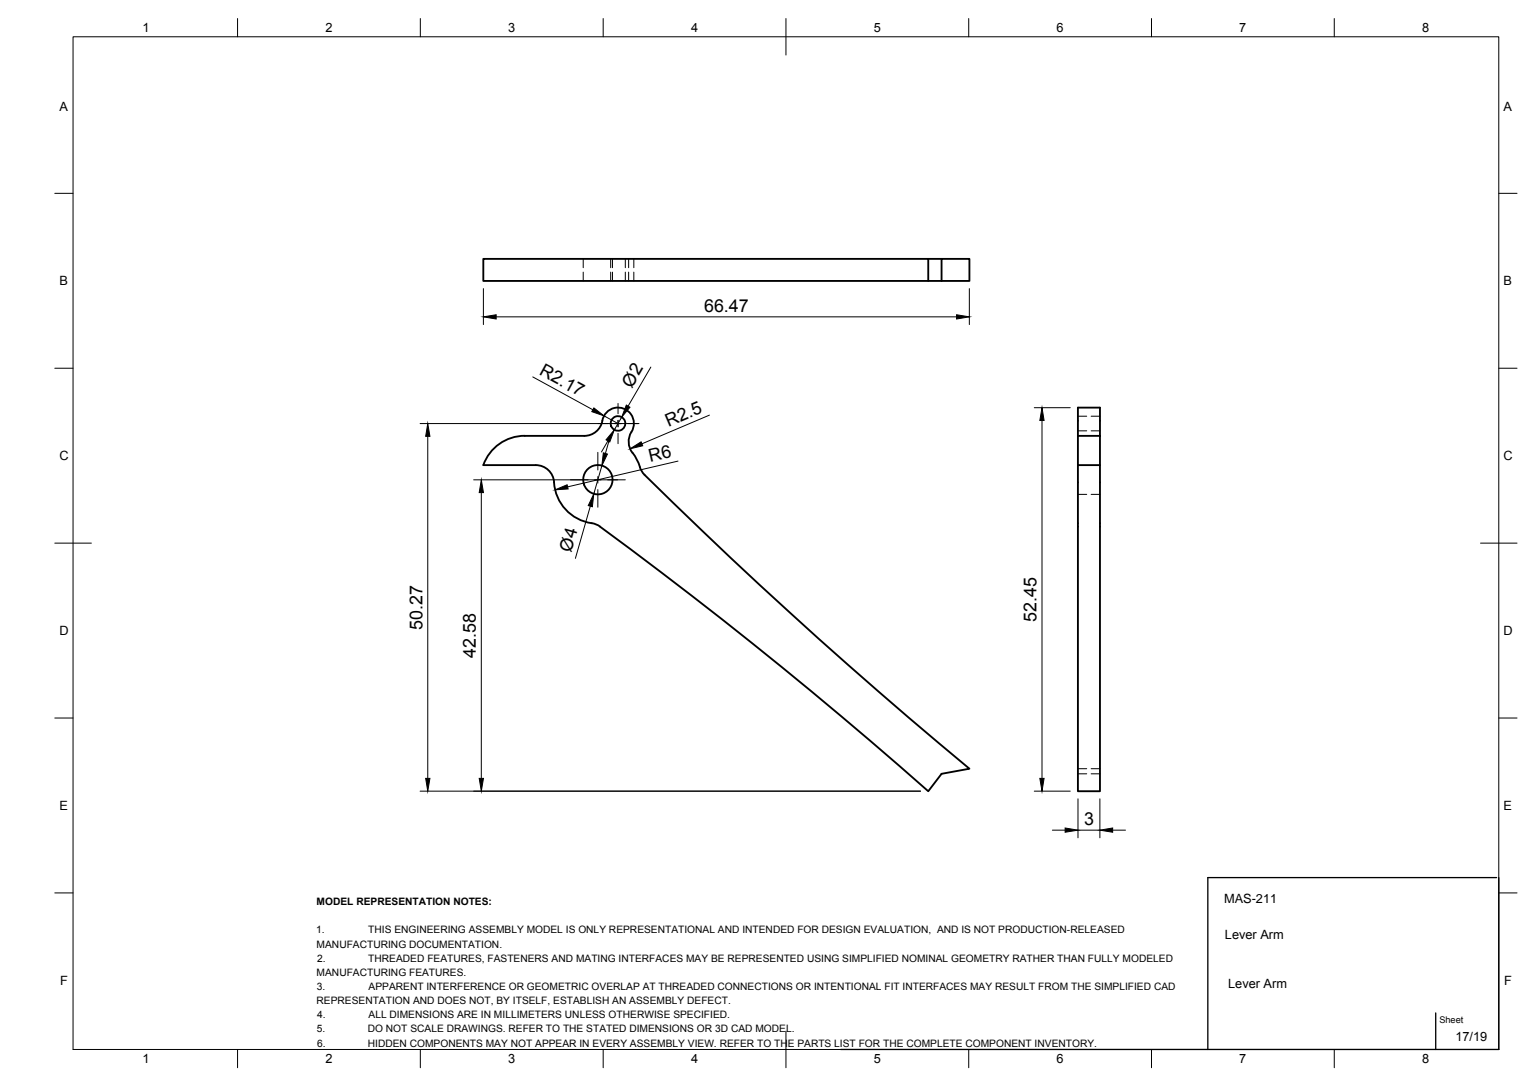
ISO-10303-21;
HEADER;
FILE_DESCRIPTION(
 (''),
 '2;1');
FILE_NAME ( 'Lever Arm.step', '2026-10-05T20:07:59+06:00', ( '' ), ( '' ), 'STEP AP214', 'Unspecified', '' );
FILE_SCHEMA (('AUTOMOTIVE_DESIGN { 1 0 10303 214 3 1 1 }'));
ENDSEC;
DATA;
#10=MECHANICAL_DESIGN_GEOMETRIC_PRESENTATION_REPRESENTATION('',(#335),#196741);
#69=(
BOUNDED_SURFACE()
B_SPLINE_SURFACE(2,1,((#194720,#194721),(#194722,#194723),(#194724,#194725)),
 .UNSPECIFIED.,.F.,.F.,.F.)
B_SPLINE_SURFACE_WITH_KNOTS((3,3),(2,2),(-66.4194892732842,-6.49328858992507),
(0.,0.36),.UNSPECIFIED.)
GEOMETRIC_REPRESENTATION_ITEM()
RATIONAL_B_SPLINE_SURFACE(((1.,1.),(0.999060551236508,0.999060551236508),
(1.,1.)))
REPRESENTATION_ITEM('')
SURFACE()
) ;
#70=(
BOUNDED_SURFACE()
B_SPLINE_SURFACE(2,1,((#194797,#194798),(#194799,#194800),(#194801,#194802)),
 .UNSPECIFIED.,.F.,.F.,.F.)
B_SPLINE_SURFACE_WITH_KNOTS((3,3),(2,2),(47.1134450647953,104.780247485259),
(0.,0.36),.UNSPECIFIED.)
GEOMETRIC_REPRESENTATION_ITEM()
RATIONAL_B_SPLINE_SURFACE(((1.,1.),(0.998981521269156,0.998981521269156),
(1.,1.)))
REPRESENTATION_ITEM('')
SURFACE()
) ;
#335=STYLED_ITEM('',(#196765),#354) ;
#354=MANIFOLD_SOLID_BREP('Lever Arm',#8731) ;
#410=PLANE('',#9042) ;
#411=PLANE('',#9060) ;
#412=PLANE('',#9064) ;
#413=PLANE('',#9076) ;
#414=PLANE('',#9083) ;
#415=PLANE('',#9084) ;
#590=FACE_BOUND('',#1605,.T.) ;
#591=FACE_BOUND('',#1606,.T.) ;
#592=FACE_BOUND('',#1608,.T.) ;
#593=FACE_BOUND('',#1609,.T.) ;
#711=CIRCLE('',#9043,691.195967278452) ;
#712=CIRCLE('',#9044,691.195967278452) ;
#713=CIRCLE('',#9046,2.49999999999962) ;
#714=CIRCLE('',#9047,2.49999999999962) ;
#715=CIRCLE('',#9049,5.99999999999934) ;
#716=CIRCLE('',#9050,5.99999999999934) ;
#717=CIRCLE('',#9052,2.50000000000002) ;
#718=CIRCLE('',#9053,2.50000000000002) ;
#719=CIRCLE('',#9055,2.17161327008905) ;
#720=CIRCLE('',#9056,2.17161327008905) ;
#721=CIRCLE('',#9058,2.50000000000002) ;
#722=CIRCLE('',#9059,2.50000000000002) ;
#723=CIRCLE('',#9062,6.00000000000005) ;
#724=CIRCLE('',#9063,6.00000000000005) ;
#725=CIRCLE('',#9066,2.49999999999997) ;
#726=CIRCLE('',#9067,2.49999999999997) ;
#727=CIRCLE('',#9069,6.00000000000009) ;
#728=CIRCLE('',#9070,6.00000000000009) ;
#729=CIRCLE('',#9072,2.50000000000032) ;
#730=CIRCLE('',#9073,2.50000000000032) ;
#731=CIRCLE('',#9074,638.804590655714) ;
#732=CIRCLE('',#9075,638.804590655714) ;
#733=CIRCLE('',#9078,2.00000000000002) ;
#734=CIRCLE('',#9079,2.00000000000002) ;
#735=CIRCLE('',#9081,1.) ;
#736=CIRCLE('',#9082,1.) ;
#1078=FACE_OUTER_BOUND('',#1587,.T.) ;
#1079=FACE_OUTER_BOUND('',#1588,.T.) ;
#1080=FACE_OUTER_BOUND('',#1589,.T.) ;
#1081=FACE_OUTER_BOUND('',#1590,.T.) ;
#1082=FACE_OUTER_BOUND('',#1591,.T.) ;
#1083=FACE_OUTER_BOUND('',#1592,.T.) ;
#1084=FACE_OUTER_BOUND('',#1593,.T.) ;
#1085=FACE_OUTER_BOUND('',#1594,.T.) ;
#1086=FACE_OUTER_BOUND('',#1595,.T.) ;
#1087=FACE_OUTER_BOUND('',#1596,.T.) ;
#1088=FACE_OUTER_BOUND('',#1597,.T.) ;
#1089=FACE_OUTER_BOUND('',#1598,.T.) ;
#1090=FACE_OUTER_BOUND('',#1599,.T.) ;
#1091=FACE_OUTER_BOUND('',#1600,.T.) ;
#1092=FACE_OUTER_BOUND('',#1601,.T.) ;
#1093=FACE_OUTER_BOUND('',#1602,.T.) ;
#1094=FACE_OUTER_BOUND('',#1603,.T.) ;
#1095=FACE_OUTER_BOUND('',#1604,.T.) ;
#1096=FACE_OUTER_BOUND('',#1607,.T.) ;
#1587=EDGE_LOOP('',(#6656,#6657,#6658,#6659)) ;
#1588=EDGE_LOOP('',(#6660,#6661,#6662,#6663)) ;
#1589=EDGE_LOOP('',(#6664,#6665,#6666,#6667)) ;
#1590=EDGE_LOOP('',(#6668,#6669,#6670,#6671)) ;
#1591=EDGE_LOOP('',(#6672,#6673,#6674,#6675)) ;
#1592=EDGE_LOOP('',(#6676,#6677,#6678,#6679)) ;
#1593=EDGE_LOOP('',(#6680,#6681,#6682,#6683)) ;
#1594=EDGE_LOOP('',(#6684,#6685,#6686,#6687)) ;
#1595=EDGE_LOOP('',(#6688,#6689,#6690,#6691)) ;
#1596=EDGE_LOOP('',(#6692,#6693,#6694,#6695)) ;
#1597=EDGE_LOOP('',(#6696,#6697,#6698,#6699)) ;
#1598=EDGE_LOOP('',(#6700,#6701,#6702,#6703)) ;
#1599=EDGE_LOOP('',(#6704,#6705,#6706,#6707)) ;
#1600=EDGE_LOOP('',(#6708,#6709,#6710,#6711)) ;
#1601=EDGE_LOOP('',(#6712,#6713,#6714,#6715)) ;
#1602=EDGE_LOOP('',(#6716,#6717,#6718,#6719)) ;
#1603=EDGE_LOOP('',(#6720,#6721,#6722,#6723)) ;
#1604=EDGE_LOOP('',(#6724,#6725,#6726,#6727,#6728,#6729,#6730,#6731,#6732,
#6733,#6734,#6735,#6736,#6737,#6738)) ;
#1605=EDGE_LOOP('',(#6739)) ;
#1606=EDGE_LOOP('',(#6740)) ;
#1607=EDGE_LOOP('',(#6741,#6742,#6743,#6744,#6745,#6746,#6747,#6748,#6749,
#6750,#6751,#6752,#6753,#6754,#6755)) ;
#1608=EDGE_LOOP('',(#6756)) ;
#1609=EDGE_LOOP('',(#6757)) ;
#2054=LINE('',#194714,#2757) ;
#2055=LINE('',#194716,#2758) ;
#2056=LINE('',#194718,#2759) ;
#2057=LINE('',#194719,#2760) ;
#2058=LINE('',#194729,#2761) ;
#2059=LINE('',#194735,#2762) ;
#2060=LINE('',#194741,#2763) ;
#2061=LINE('',#194747,#2764) ;
#2062=LINE('',#194753,#2765) ;
#2063=LINE('',#194759,#2766) ;
#2064=LINE('',#194763,#2767) ;
#2065=LINE('',#194765,#2768) ;
#2066=LINE('',#194766,#2769) ;
#2067=LINE('',#194771,#2770) ;
#2068=LINE('',#194775,#2771) ;
#2069=LINE('',#194777,#2772) ;
#2070=LINE('',#194778,#2773) ;
#2071=LINE('',#194783,#2774) ;
#2072=LINE('',#194789,#2775) ;
#2073=LINE('',#194795,#2776) ;
#2074=LINE('',#194806,#2777) ;
#2075=LINE('',#194809,#2778) ;
#2076=LINE('',#194810,#2779) ;
#2077=LINE('',#194815,#2780) ;
#2078=LINE('',#194821,#2781) ;
#2757=VECTOR('',#10240,10.) ;
#2758=VECTOR('',#10241,10.) ;
#2759=VECTOR('',#10242,10.) ;
#2760=VECTOR('',#10243,10.) ;
#2761=VECTOR('',#10246,10.) ;
#2762=VECTOR('',#10253,10.) ;
#2763=VECTOR('',#10260,10.) ;
#2764=VECTOR('',#10267,10.) ;
#2765=VECTOR('',#10274,10.) ;
#2766=VECTOR('',#10281,10.) ;
#2767=VECTOR('',#10286,10.) ;
#2768=VECTOR('',#10287,10.) ;
#2769=VECTOR('',#10288,10.) ;
#2770=VECTOR('',#10293,10.) ;
#2771=VECTOR('',#10298,10.) ;
#2772=VECTOR('',#10299,10.) ;
#2773=VECTOR('',#10300,10.) ;
#2774=VECTOR('',#10305,10.) ;
#2775=VECTOR('',#10312,10.) ;
#2776=VECTOR('',#10319,10.) ;
#2777=VECTOR('',#10324,10.) ;
#2778=VECTOR('',#10329,10.) ;
#2779=VECTOR('',#10330,10.) ;
#2780=VECTOR('',#10335,2.00000000000001) ;
#2781=VECTOR('',#10342,0.999999999999978) ;
#3804=VERTEX_POINT('',#194712) ;
#3805=VERTEX_POINT('',#194713) ;
#3806=VERTEX_POINT('',#194715) ;
#3807=VERTEX_POINT('',#194717) ;
#3808=VERTEX_POINT('',#194726) ;
#3809=VERTEX_POINT('',#194728) ;
#3810=VERTEX_POINT('',#194732) ;
#3811=VERTEX_POINT('',#194734) ;
#3812=VERTEX_POINT('',#194738) ;
#3813=VERTEX_POINT('',#194740) ;
#3814=VERTEX_POINT('',#194744) ;
#3815=VERTEX_POINT('',#194746) ;
#3816=VERTEX_POINT('',#194750) ;
#3817=VERTEX_POINT('',#194752) ;
#3818=VERTEX_POINT('',#194756) ;
#3819=VERTEX_POINT('',#194758) ;
#3820=VERTEX_POINT('',#194762) ;
#3821=VERTEX_POINT('',#194764) ;
#3822=VERTEX_POINT('',#194768) ;
#3823=VERTEX_POINT('',#194770) ;
#3824=VERTEX_POINT('',#194774) ;
#3825=VERTEX_POINT('',#194776) ;
#3826=VERTEX_POINT('',#194780) ;
#3827=VERTEX_POINT('',#194782) ;
#3828=VERTEX_POINT('',#194786) ;
#3829=VERTEX_POINT('',#194788) ;
#3830=VERTEX_POINT('',#194792) ;
#3831=VERTEX_POINT('',#194794) ;
#3832=VERTEX_POINT('',#194803) ;
#3833=VERTEX_POINT('',#194805) ;
#3834=VERTEX_POINT('',#194812) ;
#3835=VERTEX_POINT('',#194814) ;
#3836=VERTEX_POINT('',#194818) ;
#3837=VERTEX_POINT('',#194820) ;
#4836=EDGE_CURVE('',#3804,#3805,#2054,.T.) ;
#4837=EDGE_CURVE('',#3805,#3806,#2055,.T.) ;
#4838=EDGE_CURVE('',#3807,#3806,#2056,.T.) ;
#4839=EDGE_CURVE('',#3804,#3807,#2057,.T.) ;
#4840=EDGE_CURVE('',#3805,#3808,#711,.T.) ;
#4841=EDGE_CURVE('',#3808,#3809,#2058,.T.) ;
#4842=EDGE_CURVE('',#3806,#3809,#712,.T.) ;
#4843=EDGE_CURVE('',#3808,#3810,#713,.T.) ;
#4844=EDGE_CURVE('',#3810,#3811,#2059,.T.) ;
#4845=EDGE_CURVE('',#3809,#3811,#714,.T.) ;
#4846=EDGE_CURVE('',#3810,#3812,#715,.T.) ;
#4847=EDGE_CURVE('',#3812,#3813,#2060,.T.) ;
#4848=EDGE_CURVE('',#3811,#3813,#716,.T.) ;
#4849=EDGE_CURVE('',#3812,#3814,#717,.T.) ;
#4850=EDGE_CURVE('',#3814,#3815,#2061,.T.) ;
#4851=EDGE_CURVE('',#3813,#3815,#718,.T.) ;
#4852=EDGE_CURVE('',#3814,#3816,#719,.T.) ;
#4853=EDGE_CURVE('',#3816,#3817,#2062,.T.) ;
#4854=EDGE_CURVE('',#3815,#3817,#720,.T.) ;
#4855=EDGE_CURVE('',#3816,#3818,#721,.T.) ;
#4856=EDGE_CURVE('',#3818,#3819,#2063,.T.) ;
#4857=EDGE_CURVE('',#3817,#3819,#722,.T.) ;
#4858=EDGE_CURVE('',#3818,#3820,#2064,.T.) ;
#4859=EDGE_CURVE('',#3820,#3821,#2065,.T.) ;
#4860=EDGE_CURVE('',#3819,#3821,#2066,.T.) ;
#4861=EDGE_CURVE('',#3820,#3822,#723,.T.) ;
#4862=EDGE_CURVE('',#3822,#3823,#2067,.T.) ;
#4863=EDGE_CURVE('',#3821,#3823,#724,.T.) ;
#4864=EDGE_CURVE('',#3822,#3824,#2068,.T.) ;
#4865=EDGE_CURVE('',#3824,#3825,#2069,.T.) ;
#4866=EDGE_CURVE('',#3823,#3825,#2070,.T.) ;
#4867=EDGE_CURVE('',#3824,#3826,#725,.T.) ;
#4868=EDGE_CURVE('',#3826,#3827,#2071,.T.) ;
#4869=EDGE_CURVE('',#3825,#3827,#726,.T.) ;
#4870=EDGE_CURVE('',#3826,#3828,#727,.T.) ;
#4871=EDGE_CURVE('',#3828,#3829,#2072,.T.) ;
#4872=EDGE_CURVE('',#3827,#3829,#728,.T.) ;
#4873=EDGE_CURVE('',#3828,#3830,#729,.T.) ;
#4874=EDGE_CURVE('',#3830,#3831,#2073,.T.) ;
#4875=EDGE_CURVE('',#3829,#3831,#730,.T.) ;
#4876=EDGE_CURVE('',#3830,#3832,#731,.T.) ;
#4877=EDGE_CURVE('',#3832,#3833,#2074,.T.) ;
#4878=EDGE_CURVE('',#3831,#3833,#732,.T.) ;
#4879=EDGE_CURVE('',#3832,#3804,#2075,.T.) ;
#4880=EDGE_CURVE('',#3833,#3807,#2076,.T.) ;
#4881=EDGE_CURVE('',#3834,#3834,#733,.T.) ;
#4882=EDGE_CURVE('',#3834,#3835,#2077,.T.) ;
#4883=EDGE_CURVE('',#3835,#3835,#734,.T.) ;
#4884=EDGE_CURVE('',#3836,#3836,#735,.T.) ;
#4885=EDGE_CURVE('',#3836,#3837,#2078,.T.) ;
#4886=EDGE_CURVE('',#3837,#3837,#736,.T.) ;
#6656=ORIENTED_EDGE('',*,*,#4836,.T.) ;
#6657=ORIENTED_EDGE('',*,*,#4837,.T.) ;
#6658=ORIENTED_EDGE('',*,*,#4838,.F.) ;
#6659=ORIENTED_EDGE('',*,*,#4839,.F.) ;
#6660=ORIENTED_EDGE('',*,*,#4840,.T.) ;
#6661=ORIENTED_EDGE('',*,*,#4841,.T.) ;
#6662=ORIENTED_EDGE('',*,*,#4842,.F.) ;
#6663=ORIENTED_EDGE('',*,*,#4837,.F.) ;
#6664=ORIENTED_EDGE('',*,*,#4843,.T.) ;
#6665=ORIENTED_EDGE('',*,*,#4844,.T.) ;
#6666=ORIENTED_EDGE('',*,*,#4845,.F.) ;
#6667=ORIENTED_EDGE('',*,*,#4841,.F.) ;
#6668=ORIENTED_EDGE('',*,*,#4846,.T.) ;
#6669=ORIENTED_EDGE('',*,*,#4847,.T.) ;
#6670=ORIENTED_EDGE('',*,*,#4848,.F.) ;
#6671=ORIENTED_EDGE('',*,*,#4844,.F.) ;
#6672=ORIENTED_EDGE('',*,*,#4849,.T.) ;
#6673=ORIENTED_EDGE('',*,*,#4850,.T.) ;
#6674=ORIENTED_EDGE('',*,*,#4851,.F.) ;
#6675=ORIENTED_EDGE('',*,*,#4847,.F.) ;
#6676=ORIENTED_EDGE('',*,*,#4852,.T.) ;
#6677=ORIENTED_EDGE('',*,*,#4853,.T.) ;
#6678=ORIENTED_EDGE('',*,*,#4854,.F.) ;
#6679=ORIENTED_EDGE('',*,*,#4850,.F.) ;
#6680=ORIENTED_EDGE('',*,*,#4855,.T.) ;
#6681=ORIENTED_EDGE('',*,*,#4856,.T.) ;
#6682=ORIENTED_EDGE('',*,*,#4857,.F.) ;
#6683=ORIENTED_EDGE('',*,*,#4853,.F.) ;
#6684=ORIENTED_EDGE('',*,*,#4858,.T.) ;
#6685=ORIENTED_EDGE('',*,*,#4859,.T.) ;
#6686=ORIENTED_EDGE('',*,*,#4860,.F.) ;
#6687=ORIENTED_EDGE('',*,*,#4856,.F.) ;
#6688=ORIENTED_EDGE('',*,*,#4861,.T.) ;
#6689=ORIENTED_EDGE('',*,*,#4862,.T.) ;
#6690=ORIENTED_EDGE('',*,*,#4863,.F.) ;
#6691=ORIENTED_EDGE('',*,*,#4859,.F.) ;
#6692=ORIENTED_EDGE('',*,*,#4864,.T.) ;
#6693=ORIENTED_EDGE('',*,*,#4865,.T.) ;
#6694=ORIENTED_EDGE('',*,*,#4866,.F.) ;
#6695=ORIENTED_EDGE('',*,*,#4862,.F.) ;
#6696=ORIENTED_EDGE('',*,*,#4867,.T.) ;
#6697=ORIENTED_EDGE('',*,*,#4868,.T.) ;
#6698=ORIENTED_EDGE('',*,*,#4869,.F.) ;
#6699=ORIENTED_EDGE('',*,*,#4865,.F.) ;
#6700=ORIENTED_EDGE('',*,*,#4870,.T.) ;
#6701=ORIENTED_EDGE('',*,*,#4871,.T.) ;
#6702=ORIENTED_EDGE('',*,*,#4872,.F.) ;
#6703=ORIENTED_EDGE('',*,*,#4868,.F.) ;
#6704=ORIENTED_EDGE('',*,*,#4873,.T.) ;
#6705=ORIENTED_EDGE('',*,*,#4874,.T.) ;
#6706=ORIENTED_EDGE('',*,*,#4875,.F.) ;
#6707=ORIENTED_EDGE('',*,*,#4871,.F.) ;
#6708=ORIENTED_EDGE('',*,*,#4876,.T.) ;
#6709=ORIENTED_EDGE('',*,*,#4877,.T.) ;
#6710=ORIENTED_EDGE('',*,*,#4878,.F.) ;
#6711=ORIENTED_EDGE('',*,*,#4874,.F.) ;
#6712=ORIENTED_EDGE('',*,*,#4879,.T.) ;
#6713=ORIENTED_EDGE('',*,*,#4839,.T.) ;
#6714=ORIENTED_EDGE('',*,*,#4880,.F.) ;
#6715=ORIENTED_EDGE('',*,*,#4877,.F.) ;
#6716=ORIENTED_EDGE('',*,*,#4881,.F.) ;
#6717=ORIENTED_EDGE('',*,*,#4882,.T.) ;
#6718=ORIENTED_EDGE('',*,*,#4883,.T.) ;
#6719=ORIENTED_EDGE('',*,*,#4882,.F.) ;
#6720=ORIENTED_EDGE('',*,*,#4884,.F.) ;
#6721=ORIENTED_EDGE('',*,*,#4885,.T.) ;
#6722=ORIENTED_EDGE('',*,*,#4886,.T.) ;
#6723=ORIENTED_EDGE('',*,*,#4885,.F.) ;
#6724=ORIENTED_EDGE('',*,*,#4879,.F.) ;
#6725=ORIENTED_EDGE('',*,*,#4876,.F.) ;
#6726=ORIENTED_EDGE('',*,*,#4873,.F.) ;
#6727=ORIENTED_EDGE('',*,*,#4870,.F.) ;
#6728=ORIENTED_EDGE('',*,*,#4867,.F.) ;
#6729=ORIENTED_EDGE('',*,*,#4864,.F.) ;
#6730=ORIENTED_EDGE('',*,*,#4861,.F.) ;
#6731=ORIENTED_EDGE('',*,*,#4858,.F.) ;
#6732=ORIENTED_EDGE('',*,*,#4855,.F.) ;
#6733=ORIENTED_EDGE('',*,*,#4852,.F.) ;
#6734=ORIENTED_EDGE('',*,*,#4849,.F.) ;
#6735=ORIENTED_EDGE('',*,*,#4846,.F.) ;
#6736=ORIENTED_EDGE('',*,*,#4843,.F.) ;
#6737=ORIENTED_EDGE('',*,*,#4840,.F.) ;
#6738=ORIENTED_EDGE('',*,*,#4836,.F.) ;
#6739=ORIENTED_EDGE('',*,*,#4883,.F.) ;
#6740=ORIENTED_EDGE('',*,*,#4886,.F.) ;
#6741=ORIENTED_EDGE('',*,*,#4838,.T.) ;
#6742=ORIENTED_EDGE('',*,*,#4842,.T.) ;
#6743=ORIENTED_EDGE('',*,*,#4845,.T.) ;
#6744=ORIENTED_EDGE('',*,*,#4848,.T.) ;
#6745=ORIENTED_EDGE('',*,*,#4851,.T.) ;
#6746=ORIENTED_EDGE('',*,*,#4854,.T.) ;
#6747=ORIENTED_EDGE('',*,*,#4857,.T.) ;
#6748=ORIENTED_EDGE('',*,*,#4860,.T.) ;
#6749=ORIENTED_EDGE('',*,*,#4863,.T.) ;
#6750=ORIENTED_EDGE('',*,*,#4866,.T.) ;
#6751=ORIENTED_EDGE('',*,*,#4869,.T.) ;
#6752=ORIENTED_EDGE('',*,*,#4872,.T.) ;
#6753=ORIENTED_EDGE('',*,*,#4875,.T.) ;
#6754=ORIENTED_EDGE('',*,*,#4878,.T.) ;
#6755=ORIENTED_EDGE('',*,*,#4880,.T.) ;
#6756=ORIENTED_EDGE('',*,*,#4881,.T.) ;
#6757=ORIENTED_EDGE('',*,*,#4884,.T.) ;
#8194=CYLINDRICAL_SURFACE('',#9045,2.49999999999961) ;
#8195=CYLINDRICAL_SURFACE('',#9048,5.99999999999934) ;
#8196=CYLINDRICAL_SURFACE('',#9051,2.50000000000003) ;
#8197=CYLINDRICAL_SURFACE('',#9054,2.17161327008909) ;
#8198=CYLINDRICAL_SURFACE('',#9057,2.5000000000001) ;
#8199=CYLINDRICAL_SURFACE('',#9061,5.99999999999993) ;
#8200=CYLINDRICAL_SURFACE('',#9065,2.5) ;
#8201=CYLINDRICAL_SURFACE('',#9068,6.00000000000019) ;
#8202=CYLINDRICAL_SURFACE('',#9071,2.50000000000021) ;
#8203=CYLINDRICAL_SURFACE('',#9077,2.00000000000001) ;
#8204=CYLINDRICAL_SURFACE('',#9080,0.999999999999978) ;
#8461=ADVANCED_FACE('',(#1078),#410,.T.) ;
#8462=ADVANCED_FACE('',(#1079),#69,.T.) ;
#8463=ADVANCED_FACE('',(#1080),#8194,.F.) ;
#8464=ADVANCED_FACE('',(#1081),#8195,.T.) ;
#8465=ADVANCED_FACE('',(#1082),#8196,.F.) ;
#8466=ADVANCED_FACE('',(#1083),#8197,.T.) ;
#8467=ADVANCED_FACE('',(#1084),#8198,.F.) ;
#8468=ADVANCED_FACE('',(#1085),#411,.T.) ;
#8469=ADVANCED_FACE('',(#1086),#8199,.T.) ;
#8470=ADVANCED_FACE('',(#1087),#412,.T.) ;
#8471=ADVANCED_FACE('',(#1088),#8200,.F.) ;
#8472=ADVANCED_FACE('',(#1089),#8201,.T.) ;
#8473=ADVANCED_FACE('',(#1090),#8202,.F.) ;
#8474=ADVANCED_FACE('',(#1091),#70,.T.) ;
#8475=ADVANCED_FACE('',(#1092),#413,.T.) ;
#8476=ADVANCED_FACE('',(#1093),#8203,.F.) ;
#8477=ADVANCED_FACE('',(#1094),#8204,.F.) ;
#8478=ADVANCED_FACE('',(#1095,#590,#591),#414,.T.) ;
#8479=ADVANCED_FACE('',(#1096,#592,#593),#415,.T.) ;
#8731=CLOSED_SHELL('',(#8461,#8462,#8463,#8464,#8465,#8466,#8467,#8468,
#8469,#8470,#8471,#8472,#8473,#8474,#8475,#8476,#8477,#8478,#8479)) ;
#9042=AXIS2_PLACEMENT_3D('',#194711,#10238,#10239) ;
#9043=AXIS2_PLACEMENT_3D('',#194727,#10244,#10245) ;
#9044=AXIS2_PLACEMENT_3D('',#194730,#10247,#10248) ;
#9045=AXIS2_PLACEMENT_3D('',#194731,#10249,#10250) ;
#9046=AXIS2_PLACEMENT_3D('',#194733,#10251,#10252) ;
#9047=AXIS2_PLACEMENT_3D('',#194736,#10254,#10255) ;
#9048=AXIS2_PLACEMENT_3D('',#194737,#10256,#10257) ;
#9049=AXIS2_PLACEMENT_3D('',#194739,#10258,#10259) ;
#9050=AXIS2_PLACEMENT_3D('',#194742,#10261,#10262) ;
#9051=AXIS2_PLACEMENT_3D('',#194743,#10263,#10264) ;
#9052=AXIS2_PLACEMENT_3D('',#194745,#10265,#10266) ;
#9053=AXIS2_PLACEMENT_3D('',#194748,#10268,#10269) ;
#9054=AXIS2_PLACEMENT_3D('',#194749,#10270,#10271) ;
#9055=AXIS2_PLACEMENT_3D('',#194751,#10272,#10273) ;
#9056=AXIS2_PLACEMENT_3D('',#194754,#10275,#10276) ;
#9057=AXIS2_PLACEMENT_3D('',#194755,#10277,#10278) ;
#9058=AXIS2_PLACEMENT_3D('',#194757,#10279,#10280) ;
#9059=AXIS2_PLACEMENT_3D('',#194760,#10282,#10283) ;
#9060=AXIS2_PLACEMENT_3D('',#194761,#10284,#10285) ;
#9061=AXIS2_PLACEMENT_3D('',#194767,#10289,#10290) ;
#9062=AXIS2_PLACEMENT_3D('',#194769,#10291,#10292) ;
#9063=AXIS2_PLACEMENT_3D('',#194772,#10294,#10295) ;
#9064=AXIS2_PLACEMENT_3D('',#194773,#10296,#10297) ;
#9065=AXIS2_PLACEMENT_3D('',#194779,#10301,#10302) ;
#9066=AXIS2_PLACEMENT_3D('',#194781,#10303,#10304) ;
#9067=AXIS2_PLACEMENT_3D('',#194784,#10306,#10307) ;
#9068=AXIS2_PLACEMENT_3D('',#194785,#10308,#10309) ;
#9069=AXIS2_PLACEMENT_3D('',#194787,#10310,#10311) ;
#9070=AXIS2_PLACEMENT_3D('',#194790,#10313,#10314) ;
#9071=AXIS2_PLACEMENT_3D('',#194791,#10315,#10316) ;
#9072=AXIS2_PLACEMENT_3D('',#194793,#10317,#10318) ;
#9073=AXIS2_PLACEMENT_3D('',#194796,#10320,#10321) ;
#9074=AXIS2_PLACEMENT_3D('',#194804,#10322,#10323) ;
#9075=AXIS2_PLACEMENT_3D('',#194807,#10325,#10326) ;
#9076=AXIS2_PLACEMENT_3D('',#194808,#10327,#10328) ;
#9077=AXIS2_PLACEMENT_3D('',#194811,#10331,#10332) ;
#9078=AXIS2_PLACEMENT_3D('',#194813,#10333,#10334) ;
#9079=AXIS2_PLACEMENT_3D('',#194816,#10336,#10337) ;
#9080=AXIS2_PLACEMENT_3D('',#194817,#10338,#10339) ;
#9081=AXIS2_PLACEMENT_3D('',#194819,#10340,#10341) ;
#9082=AXIS2_PLACEMENT_3D('',#194822,#10343,#10344) ;
#9083=AXIS2_PLACEMENT_3D('',#194823,#10345,#10346) ;
#9084=AXIS2_PLACEMENT_3D('',#194824,#10347,#10348) ;
#10238=DIRECTION('center_axis',(0.148915206578323,0.,-0.988849969029547)) ;
#10239=DIRECTION('ref_axis',(-0.988849969029547,0.,-0.148915206578323)) ;
#10240=DIRECTION('',(-0.988849969029547,0.,-0.148915206578323)) ;
#10241=DIRECTION('',(0.,1.,0.)) ;
#10242=DIRECTION('',(-0.988849969029547,0.,-0.148915206578323)) ;
#10243=DIRECTION('',(0.,1.,0.)) ;
#10244=DIRECTION('center_axis',(-1.08830637864895E-26,-1.,6.02632521955549E-27)) ;
#10245=DIRECTION('ref_axis',(0.895004054636058,-1.24231708851682E-26,-0.446058003162163)) ;
#10246=DIRECTION('',(0.,1.,0.)) ;
#10247=DIRECTION('center_axis',(-7.47878448692068E-16,-1.,4.14125915728814E-16)) ;
#10248=DIRECTION('ref_axis',(0.895004054636058,-8.5371380263067E-16,-0.446058003162163)) ;
#10249=DIRECTION('center_axis',(0.,1.,0.)) ;
#10250=DIRECTION('ref_axis',(0.97735290249656,0.,-0.211615935084173)) ;
#10251=DIRECTION('center_axis',(0.,-1.,0.)) ;
#10252=DIRECTION('ref_axis',(0.999355666138518,0.,0.0358922353279835)) ;
#10253=DIRECTION('',(0.,1.,0.)) ;
#10254=DIRECTION('center_axis',(0.,-1.,0.)) ;
#10255=DIRECTION('ref_axis',(0.999355666138518,0.,0.0358922353279835)) ;
#10256=DIRECTION('center_axis',(0.,-1.,0.)) ;
#10257=DIRECTION('ref_axis',(-0.989177166167747,0.,0.146726050626141)) ;
#10258=DIRECTION('center_axis',(0.,1.,0.)) ;
#10259=DIRECTION('ref_axis',(-0.945907682666056,0.,0.324435904106393)) ;
#10260=DIRECTION('',(0.,1.,0.)) ;
#10261=DIRECTION('center_axis',(0.,1.,0.)) ;
#10262=DIRECTION('ref_axis',(-0.945907682666056,0.,0.324435904106393)) ;
#10263=DIRECTION('center_axis',(0.,1.,0.)) ;
#10264=DIRECTION('ref_axis',(0.961183535222693,0.,0.275909788910806)) ;
#10265=DIRECTION('center_axis',(-1.72231588589536E-26,-1.,-4.94394457563211E-27)) ;
#10266=DIRECTION('ref_axis',(0.629810177126175,-1.61558713389262E-26,0.776749084832609)) ;
#10267=DIRECTION('',(0.,1.,0.)) ;
#10268=DIRECTION('center_axis',(0.,-1.,0.)) ;
#10269=DIRECTION('ref_axis',(0.629810177126175,0.,0.776749084832609)) ;
#10270=DIRECTION('center_axis',(0.,-1.,0.)) ;
#10271=DIRECTION('ref_axis',(-0.641485626683685,0.,0.767135053793163)) ;
#10272=DIRECTION('center_axis',(0.,1.,0.)) ;
#10273=DIRECTION('ref_axis',(0.875957545458479,0.,0.482388203166658)) ;
#10274=DIRECTION('',(0.,1.,0.)) ;
#10275=DIRECTION('center_axis',(0.,1.,0.)) ;
#10276=DIRECTION('ref_axis',(0.875957545458479,0.,0.482388203166658)) ;
#10277=DIRECTION('center_axis',(0.,1.,0.)) ;
#10278=DIRECTION('ref_axis',(-0.360497640279418,0.,-0.932760125301769)) ;
#10279=DIRECTION('center_axis',(0.,-1.,0.)) ;
#10280=DIRECTION('ref_axis',(0.323867587736058,0.,-0.94610241814194)) ;
#10281=DIRECTION('',(0.,1.,0.)) ;
#10282=DIRECTION('center_axis',(3.41689582144301E-16,-1.,8.84095710607688E-16)) ;
#10283=DIRECTION('ref_axis',(0.323867587736058,-6.66133814775089E-16,-0.94610241814194)) ;
#10284=DIRECTION('center_axis',(-0.323867587736067,0.,0.946102418141937)) ;
#10285=DIRECTION('ref_axis',(0.946102418141937,0.,0.323867587736067)) ;
#10286=DIRECTION('',(0.946102418141937,0.,0.323867587736067)) ;
#10287=DIRECTION('',(0.,1.,0.)) ;
#10288=DIRECTION('',(0.946102418141937,0.,0.323867587736067)) ;
#10289=DIRECTION('center_axis',(0.,-1.,0.)) ;
#10290=DIRECTION('ref_axis',(0.281795707735394,0.,0.959474428581559)) ;
#10291=DIRECTION('center_axis',(0.,1.,0.)) ;
#10292=DIRECTION('ref_axis',(0.78403805150818,0.,0.620712762706919)) ;
#10293=DIRECTION('',(0.,1.,0.)) ;
#10294=DIRECTION('center_axis',(1.42075501258625E-16,1.,4.83746936676411E-16)) ;
#10295=DIRECTION('ref_axis',(0.78403805150818,-3.70074341541716E-16,0.620712762706919)) ;
#10296=DIRECTION('center_axis',(0.323867587736072,0.,-0.946102418141936)) ;
#10297=DIRECTION('ref_axis',(-0.946102418141936,0.,-0.323867587736072)) ;
#10298=DIRECTION('',(-0.946102418141936,0.,-0.323867587736072)) ;
#10299=DIRECTION('',(0.,1.,0.)) ;
#10300=DIRECTION('',(-0.946102418141936,0.,-0.323867587736072)) ;
#10301=DIRECTION('center_axis',(0.,1.,0.)) ;
#10302=DIRECTION('ref_axis',(-0.884669187906721,0.,0.466219291716315)) ;
#10303=DIRECTION('center_axis',(0.,-1.,0.)) ;
#10304=DIRECTION('ref_axis',(-0.963515178899987,0.,-0.267653694219464)) ;
#10305=DIRECTION('',(0.,1.,0.)) ;
#10306=DIRECTION('center_axis',(0.,-1.,0.)) ;
#10307=DIRECTION('ref_axis',(-0.963515178899987,0.,-0.267653694219464)) ;
#10308=DIRECTION('center_axis',(0.,-1.,0.)) ;
#10309=DIRECTION('ref_axis',(0.915016641398165,0.,-0.403416095321471)) ;
#10310=DIRECTION('center_axis',(5.44264897655763E-27,1.,-2.39957624702134E-27)) ;
#10311=DIRECTION('ref_axis',(0.452302175480044,-4.03896783473152E-27,-0.89186475547362)) ;
#10312=DIRECTION('',(0.,1.,0.)) ;
#10313=DIRECTION('center_axis',(0.,1.,0.)) ;
#10314=DIRECTION('ref_axis',(0.452302175480044,0.,-0.89186475547362)) ;
#10315=DIRECTION('center_axis',(0.,1.,0.)) ;
#10316=DIRECTION('ref_axis',(-0.65655456191829,0.,0.754278534245992)) ;
#10317=DIRECTION('center_axis',(0.,-1.,0.)) ;
#10318=DIRECTION('ref_axis',(-0.820987567029615,0.,0.570946069942506)) ;
#10319=DIRECTION('',(0.,1.,0.)) ;
#10320=DIRECTION('center_axis',(0.,-1.,0.)) ;
#10321=DIRECTION('ref_axis',(-0.820987567029615,0.,0.570946069942506)) ;
#10322=DIRECTION('center_axis',(2.10056525288621E-26,-1.,-1.32433786101226E-26)) ;
#10323=DIRECTION('ref_axis',(-0.869115672797272,-2.48102628179586E-26,0.494608883157335)) ;
#10324=DIRECTION('',(0.,1.,0.)) ;
#10325=DIRECTION('center_axis',(0.,-1.,0.)) ;
#10326=DIRECTION('ref_axis',(-0.869115672797272,0.,0.494608883157335)) ;
#10327=DIRECTION('center_axis',(-0.554110366789135,0.,-0.832443212127296)) ;
#10328=DIRECTION('ref_axis',(-0.832443212127296,0.,0.554110366789135)) ;
#10329=DIRECTION('',(-0.832443212127296,0.,0.554110366789135)) ;
#10330=DIRECTION('',(-0.832443212127296,0.,0.554110366789135)) ;
#10331=DIRECTION('center_axis',(0.,1.,0.)) ;
#10332=DIRECTION('ref_axis',(-0.519132143162002,0.,-0.854693990815442)) ;
#10333=DIRECTION('center_axis',(4.61307474394722E-16,-1.,-2.01875545076625E-16)) ;
#10334=DIRECTION('ref_axis',(0.919153266546442,2.77555756156287E-16,0.393900079457984)) ;
#10335=DIRECTION('',(0.,-1.,0.)) ;
#10336=DIRECTION('center_axis',(1.56231020031328E-27,-1.,1.35626158679747E-27)) ;
#10337=DIRECTION('ref_axis',(0.919153266546442,0.,0.393900079457984)) ;
#10338=DIRECTION('center_axis',(0.,1.,0.)) ;
#10339=DIRECTION('ref_axis',(-0.99990130540252,0.,0.0140491798457102)) ;
#10340=DIRECTION('center_axis',(0.,-1.,0.)) ;
#10341=DIRECTION('ref_axis',(0.805581616852069,0.,-0.592484817181003)) ;
#10342=DIRECTION('',(0.,-1.,0.)) ;
#10343=DIRECTION('center_axis',(-3.92234304386299E-27,-1.,1.31767206146335E-27)) ;
#10344=DIRECTION('ref_axis',(0.805581616852069,0.,-0.592484817181003)) ;
#10345=DIRECTION('center_axis',(0.,-1.,0.)) ;
#10346=DIRECTION('ref_axis',(0.,0.,-1.)) ;
#10347=DIRECTION('center_axis',(0.,1.,0.)) ;
#10348=DIRECTION('ref_axis',(0.,0.,1.)) ;
#194711=CARTESIAN_POINT('Origin',(-62.2357882624759,4.95951629533962E-11,
66.631932161929)) ;
#194712=CARTESIAN_POINT('',(-60.3236060552914,4.95951629533962E-11,66.91989597577)) ;
#194713=CARTESIAN_POINT('',(-64.1479704696604,4.95951629533962E-11,66.343968348088)) ;
#194714=CARTESIAN_POINT('',(-60.3236060552914,4.95951629533962E-11,66.91989597577)) ;
#194715=CARTESIAN_POINT('',(-64.1479704696604,3.00000000004959,66.343968348088)) ;
#194716=CARTESIAN_POINT('',(-64.1479704696604,4.95951629533962E-11,66.343968348088)) ;
#194717=CARTESIAN_POINT('',(-60.3236060552914,3.00000000004959,66.91989597577)) ;
#194718=CARTESIAN_POINT('',(-60.3236060552914,3.00000000004959,66.91989597577)) ;
#194719=CARTESIAN_POINT('',(-60.3236060552914,4.95951629533962E-11,66.91989597577)) ;
#194720=CARTESIAN_POINT('Ctrl Pts',(-64.1479704696604,4.95951629533962E-11,
66.343968348088)) ;
#194721=CARTESIAN_POINT('Ctrl Pts',(-64.1479704696604,3.6000000000496,66.343968348088)) ;
#194722=CARTESIAN_POINT('Ctrl Pts',(-48.5009761261745,4.95951629533962E-11,
91.9190517712764)) ;
#194723=CARTESIAN_POINT('Ctrl Pts',(-48.5009761261745,3.6000000000496,91.9190517712764)) ;
#194724=CARTESIAN_POINT('Ctrl Pts',(-35.1273171461558,4.95951629533962E-11,
118.752958858659)) ;
#194725=CARTESIAN_POINT('Ctrl Pts',(-35.1273171461558,3.6000000000496,118.752958858659)) ;
#194726=CARTESIAN_POINT('',(-35.1273171461558,4.95951629533962E-11,118.752958858659)) ;
#194727=CARTESIAN_POINT('Origin',(-653.750510408462,4.95951629534048E-11,
427.066451816625)) ;
#194728=CARTESIAN_POINT('',(-35.1273171461558,3.00000000004959,118.752958858659)) ;
#194729=CARTESIAN_POINT('',(-35.1273171461558,4.95951629533962E-11,118.752958858659)) ;
#194730=CARTESIAN_POINT('Origin',(-653.750510408462,3.00000000005019,427.066451816625)) ;
#194731=CARTESIAN_POINT('Origin',(-37.3648272827455,4.95951629533962E-11,
119.868103866564)) ;
#194732=CARTESIAN_POINT('',(-34.8664381173996,4.95951629533962E-11,119.957834454884)) ;
#194733=CARTESIAN_POINT('Origin',(-37.3648272827455,4.95951629533962E-11,
119.868103866564)) ;
#194734=CARTESIAN_POINT('',(-34.8664381173996,3.00000000004959,119.957834454884)) ;
#194735=CARTESIAN_POINT('',(-34.8664381173996,4.95951629533962E-11,119.957834454884)) ;
#194736=CARTESIAN_POINT('Origin',(-37.3648272827455,3.00000000004959,119.868103866564)) ;
#194737=CARTESIAN_POINT('Origin',(-28.8703041205692,4.95951629533962E-11,
120.173187866852)) ;
#194738=CARTESIAN_POINT('',(-34.5457502165649,4.95951629533962E-11,122.11980329149)) ;
#194739=CARTESIAN_POINT('Origin',(-28.8703041205692,4.95951629533962E-11,
120.173187866852)) ;
#194740=CARTESIAN_POINT('',(-34.5457502165649,3.00000000004959,122.11980329149)) ;
#194741=CARTESIAN_POINT('',(-34.5457502165649,4.95951629533962E-11,122.11980329149)) ;
#194742=CARTESIAN_POINT('Origin',(-28.8703041205692,3.00000000004959,120.173187866852)) ;
#194743=CARTESIAN_POINT('Origin',(-36.9105194232301,4.95951629533962E-11,
122.930893051756)) ;
#194744=CARTESIAN_POINT('',(-35.3359939804146,4.95951629533962E-11,124.872765763838)) ;
#194745=CARTESIAN_POINT('Origin',(-36.9105194232301,4.95951629533962E-11,
122.930893051756)) ;
#194746=CARTESIAN_POINT('',(-35.3359939804146,3.00000000004959,124.872765763838)) ;
#194747=CARTESIAN_POINT('',(-35.3359939804146,4.95951629533962E-11,124.872765763838)) ;
#194748=CARTESIAN_POINT('Origin',(-36.9105194232301,3.00000000004959,122.930893051756)) ;
#194749=CARTESIAN_POINT('Origin',(-33.9682898421302,4.95951629533962E-11,
126.55956438399)) ;
#194750=CARTESIAN_POINT('',(-32.066048812378,4.95951629533962E-11,127.607125007321)) ;
#194751=CARTESIAN_POINT('Origin',(-33.9682898421302,4.95951629533962E-11,
126.55956438399)) ;
#194752=CARTESIAN_POINT('',(-32.066048812378,3.00000000004959,127.607125007321)) ;
#194753=CARTESIAN_POINT('',(-32.066048812378,4.95951629533962E-11,127.607125007321)) ;
#194754=CARTESIAN_POINT('Origin',(-33.9682898421302,3.00000000004959,126.55956438399)) ;
#194755=CARTESIAN_POINT('Origin',(-29.8761549487317,4.95951629533962E-11,
128.813095515238)) ;
#194756=CARTESIAN_POINT('',(-29.0664859793916,4.95951629533962E-11,126.447839469883)) ;
#194757=CARTESIAN_POINT('Origin',(-29.8761549487317,4.95951629533962E-11,
128.813095515238)) ;
#194758=CARTESIAN_POINT('',(-29.0664859793916,3.00000000004959,126.447839469883)) ;
#194759=CARTESIAN_POINT('',(-29.0664859793916,4.95951629533962E-11,126.447839469883)) ;
#194760=CARTESIAN_POINT('Origin',(-29.8761549487317,3.0000000000496,128.813095515238)) ;
#194761=CARTESIAN_POINT('Origin',(-25.2094857224778,4.95951629533962E-11,
127.768158861474)) ;
#194762=CARTESIAN_POINT('',(-21.3524854655639,4.95951629533962E-11,129.088478253065)) ;
#194763=CARTESIAN_POINT('',(-29.0664859793916,4.95951629533962E-11,126.447839469883)) ;
#194764=CARTESIAN_POINT('',(-21.3524854655639,3.00000000004959,129.088478253065)) ;
#194765=CARTESIAN_POINT('',(-21.3524854655639,4.95951629533962E-11,129.088478253065)) ;
#194766=CARTESIAN_POINT('',(-29.0664859793916,3.00000000004959,126.447839469883)) ;
#194767=CARTESIAN_POINT('Origin',(-19.4092799391475,4.95951629533962E-11,
123.411863744214)) ;
#194768=CARTESIAN_POINT('',(-14.7050516300984,4.95951629533962E-11,127.136140320455)) ;
#194769=CARTESIAN_POINT('Origin',(-19.4092799391475,4.95951629533962E-11,
123.411863744213)) ;
#194770=CARTESIAN_POINT('',(-14.7050516300984,3.00000000004959,127.136140320455)) ;
#194771=CARTESIAN_POINT('',(-14.7050516300984,4.95951629533962E-11,127.136140320455)) ;
#194772=CARTESIAN_POINT('Origin',(-19.4092799391475,3.0000000000496,123.411863744213)) ;
#194773=CARTESIAN_POINT('Origin',(-18.0975728496786,4.95951629533962E-11,
125.974820316764)) ;
#194774=CARTESIAN_POINT('',(-21.4900940692588,4.95951629533962E-11,124.813500313073)) ;
#194775=CARTESIAN_POINT('',(-14.7050516300984,4.95951629533962E-11,127.136140320455)) ;
#194776=CARTESIAN_POINT('',(-21.4900940692588,3.00000000004959,124.813500313073)) ;
#194777=CARTESIAN_POINT('',(-21.4900940692588,4.95951629533962E-11,124.813500313073)) ;
#194778=CARTESIAN_POINT('',(-14.7050516300984,3.00000000004959,127.136140320455)) ;
#194779=CARTESIAN_POINT('Origin',(-20.6804250999186,4.95951629533962E-11,
122.448244267718)) ;
#194780=CARTESIAN_POINT('',(-23.0892130471686,4.95951629533962E-11,121.779110032169)) ;
#194781=CARTESIAN_POINT('Origin',(-20.6804250999186,4.95951629533962E-11,
122.448244267718)) ;
#194782=CARTESIAN_POINT('',(-23.0892130471686,3.00000000004959,121.779110032169)) ;
#194783=CARTESIAN_POINT('',(-23.0892130471686,4.95951629533962E-11,121.779110032169)) ;
#194784=CARTESIAN_POINT('Origin',(-20.6804250999186,3.00000000004959,122.448244267718)) ;
#194785=CARTESIAN_POINT('Origin',(-28.8703041205687,4.95951629533962E-11,
120.173187866852)) ;
#194786=CARTESIAN_POINT('',(-26.1564910676883,4.95951629533962E-11,114.82199933401)) ;
#194787=CARTESIAN_POINT('Origin',(-28.8703041205686,4.95951629533962E-11,
120.173187866852)) ;
#194788=CARTESIAN_POINT('',(-26.1564910676883,3.00000000004959,114.82199933401)) ;
#194789=CARTESIAN_POINT('',(-26.1564910676883,4.95951629533962E-11,114.82199933401)) ;
#194790=CARTESIAN_POINT('Origin',(-28.8703041205686,3.00000000004959,120.173187866852)) ;
#194791=CARTESIAN_POINT('Origin',(-25.0257356289886,4.95951629533962E-11,
112.592337445326)) ;
#194792=CARTESIAN_POINT('',(-27.0782045465628,4.95951629533962E-11,114.019702620182)) ;
#194793=CARTESIAN_POINT('Origin',(-25.0257356289885,4.95951629533962E-11,
112.592337445326)) ;
#194794=CARTESIAN_POINT('',(-27.0782045465628,3.00000000004959,114.019702620182)) ;
#194795=CARTESIAN_POINT('',(-27.0782045465628,4.95951629533962E-11,114.019702620182)) ;
#194796=CARTESIAN_POINT('Origin',(-25.0257356289885,3.00000000004959,112.592337445326)) ;
#194797=CARTESIAN_POINT('Ctrl Pts',(-27.0782045465628,4.95951629533962E-11,
114.019702620182)) ;
#194798=CARTESIAN_POINT('Ctrl Pts',(-27.0782045465628,3.6000000000496,114.019702620182)) ;
#194799=CARTESIAN_POINT('Ctrl Pts',(-43.5517103463888,4.95951629533962E-11,
90.3317500112603)) ;
#194800=CARTESIAN_POINT('Ctrl Pts',(-43.5517103463888,3.6000000000496,90.3317500112603)) ;
#194801=CARTESIAN_POINT('Ctrl Pts',(-57.8226594504937,4.95951629533962E-11,
65.2551572640889)) ;
#194802=CARTESIAN_POINT('Ctrl Pts',(-57.8226594504937,3.6000000000496,65.2551572640889)) ;
#194803=CARTESIAN_POINT('',(-57.8226594504937,4.95951629533962E-11,65.2551572640889)) ;
#194804=CARTESIAN_POINT('Origin',(497.372422143233,4.9595162953412E-11,
-250.703267875912)) ;
#194805=CARTESIAN_POINT('',(-57.8226594504937,3.00000000004959,65.2551572640889)) ;
#194806=CARTESIAN_POINT('',(-57.8226594504937,4.95951629533962E-11,65.2551572640889)) ;
#194807=CARTESIAN_POINT('Origin',(497.372422143233,3.00000000004959,-250.703267875912)) ;
#194808=CARTESIAN_POINT('Origin',(-59.0731327528925,4.95951629533962E-11,
66.0875266199294)) ;
#194809=CARTESIAN_POINT('',(-57.8226594504937,4.95951629533962E-11,65.2551572640889)) ;
#194810=CARTESIAN_POINT('',(-57.8226594504937,3.00000000004959,65.2551572640889)) ;
#194811=CARTESIAN_POINT('Origin',(-28.8703041205685,4.95951629533962E-11,
120.173187866852)) ;
#194812=CARTESIAN_POINT('',(-27.8320398342445,3.00000000004959,121.882575848483)) ;
#194813=CARTESIAN_POINT('Origin',(-28.8703041205685,3.00000000004959,120.173187866852)) ;
#194814=CARTESIAN_POINT('',(-27.8320398342445,4.95951629533962E-11,121.882575848483)) ;
#194815=CARTESIAN_POINT('',(-27.8320398342445,4.95951629533962E-11,121.882575848483)) ;
#194816=CARTESIAN_POINT('Origin',(-28.8703041205685,4.95951629533962E-11,
120.173187866852)) ;
#194817=CARTESIAN_POINT('Origin',(-33.9682898421303,4.95951629533962E-11,
126.55956438399)) ;
#194818=CARTESIAN_POINT('',(-32.9683885367277,3.00000000004959,126.545515204144)) ;
#194819=CARTESIAN_POINT('Origin',(-33.9682898421302,3.00000000004959,126.55956438399)) ;
#194820=CARTESIAN_POINT('',(-32.9683885367277,4.95951629533962E-11,126.545515204144)) ;
#194821=CARTESIAN_POINT('',(-32.9683885367278,4.95951629533962E-11,126.545515204144)) ;
#194822=CARTESIAN_POINT('Origin',(-33.9682898421302,4.95951629533962E-11,
126.55956438399)) ;
#194823=CARTESIAN_POINT('Origin',(-27.8320398342445,4.95951629533962E-11,
121.882575848483)) ;
#194824=CARTESIAN_POINT('Origin',(-27.8320398342445,3.00000000004959,121.882575848483)) ;
#196737=UNCERTAINTY_MEASURE_WITH_UNIT(LENGTH_MEASURE(0.01),#196742,
'DISTANCE_ACCURACY_VALUE',
'Maximum model space distance between geometric entities at asserted c
onnectivities') ;
#196738=UNCERTAINTY_MEASURE_WITH_UNIT(LENGTH_MEASURE(0.01),#196742,
'DISTANCE_ACCURACY_VALUE',
'Maximum model space distance between geometric entities at asserted c
onnectivities') ;
#196740=(
GEOMETRIC_REPRESENTATION_CONTEXT(3)
GLOBAL_UNCERTAINTY_ASSIGNED_CONTEXT((#196737))
GLOBAL_UNIT_ASSIGNED_CONTEXT((#196742,#196744,#196745))
REPRESENTATION_CONTEXT('','3D')
) ;
#196741=(
GEOMETRIC_REPRESENTATION_CONTEXT(3)
GLOBAL_UNCERTAINTY_ASSIGNED_CONTEXT((#196738))
GLOBAL_UNIT_ASSIGNED_CONTEXT((#196742,#196744,#196745))
REPRESENTATION_CONTEXT('','3D')
) ;
#196742=(
LENGTH_UNIT()
NAMED_UNIT(*)
SI_UNIT(.MILLI.,.METRE.)
) ;
#196744=(
NAMED_UNIT(*)
PLANE_ANGLE_UNIT()
SI_UNIT($,.RADIAN.)
) ;
#196745=(
NAMED_UNIT(*)
SI_UNIT($,.STERADIAN.)
SOLID_ANGLE_UNIT()
) ;
#196753=PRODUCT_DEFINITION_CONTEXT('part definition',#196761,'design') ;
#196761=APPLICATION_CONTEXT(
'Core Data for Automotive Mechanical Design Process') ;
#196762=PRODUCT_CONTEXT('part definition',#196761,'mechanical') ;
#196765=PRESENTATION_STYLE_ASSIGNMENT((#196767)) ;
#196767=SURFACE_STYLE_USAGE(.BOTH.,#196769) ;
#196769=SURFACE_SIDE_STYLE('',(#196771)) ;
#196771=SURFACE_STYLE_FILL_AREA(#196773) ;
#196773=FILL_AREA_STYLE('Steel - Satin',(#196775)) ;
#196775=FILL_AREA_STYLE_COLOUR('Steel - Satin',#196777) ;
#196777=COLOUR_RGB('Steel - Satin', 0.09019608, 0.27058824, 0.51372549) ;
#197163=CARTESIAN_POINT ( '', ( 0.0, 0.0, 0.0 ) ) ;
#197164=DIRECTION ( '', ( 0.0, 0.0, 1.0 ) ) ;
#197165=DIRECTION ( '', ( 1.0, 0.0, 0.0 ) ) ;
#197166=AXIS2_PLACEMENT_3D ( '', #197163, #197164, #197165 ) ;
#197167=ADVANCED_BREP_SHAPE_REPRESENTATION ( 'Lever Arm', ( #354, #197166, #197177, #197446 ), #196740 ) ;
#197168=PRODUCT( 'Lever Arm', 'Lever Arm', '', ( #196762 ) ) ;
#197169=PRODUCT_DEFINITION_FORMATION ( '', '', #197168 ) ;
#197170=PRODUCT_DEFINITION( 'Lever Arm', 'Lever Arm', #197169, #196753 ) ;
#197171=PRODUCT_DEFINITION_SHAPE ( '', '', #197170 ) ;
#197172=SHAPE_DEFINITION_REPRESENTATION ( #197171, #197167 ) ;
#197174=CARTESIAN_POINT ( '', ( 0.0, 0.0, 0.0 ) ) ;
#197175=DIRECTION ( '', ( 0.0, 0.0, 1.0 ) ) ;
#197176=DIRECTION ( '', ( 1.0, 0.0, 0.0 ) ) ;
#197177=AXIS2_PLACEMENT_3D ( '', #197174, #197175, #197176 ) ;
#197443=CARTESIAN_POINT ( '', ( 0.0, 0.0, 0.0 ) ) ;
#197444=DIRECTION ( '', ( 0.0, 0.0, 1.0 ) ) ;
#197445=DIRECTION ( '', ( 1.0, 0.0, 0.0 ) ) ;
#197446=AXIS2_PLACEMENT_3D ( '', #197443, #197444, #197445 ) ;
ENDSEC;
END-ISO-10303-21;
